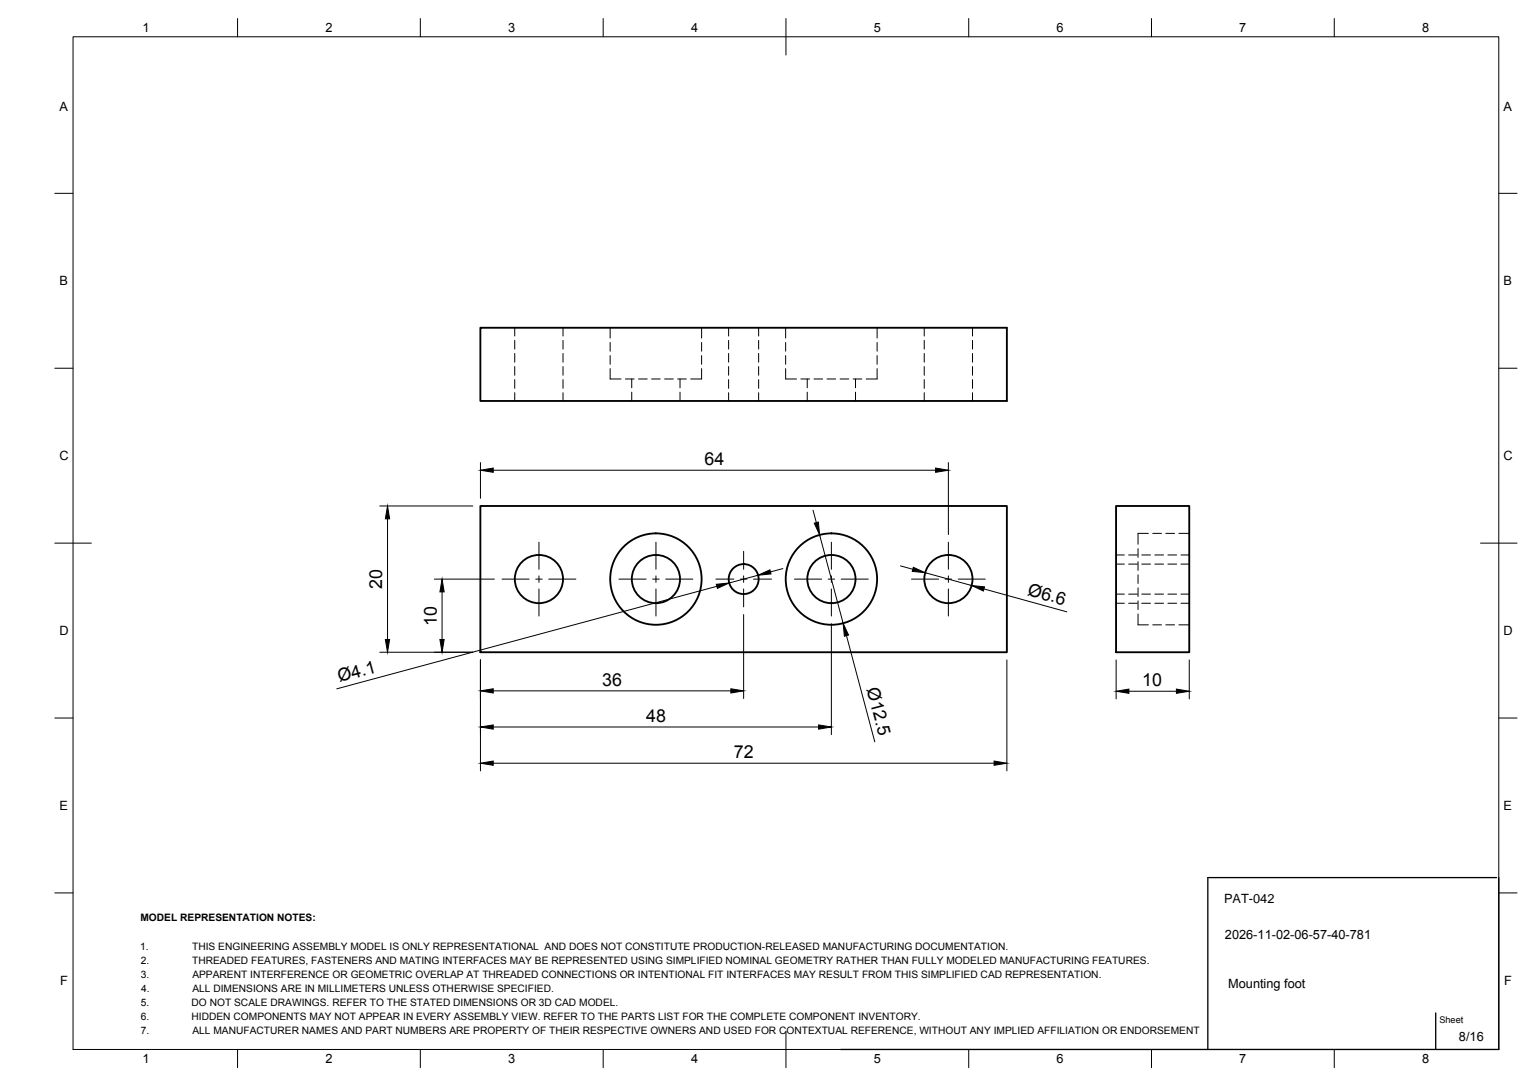
ISO-10303-21;
HEADER;
/* Generated by software containing ST-Developer
 * from STEP Tools, Inc. (www.steptools.com) 
 */

FILE_DESCRIPTION(
/* description */ ('Manifold and mounting hardware'),
/* implementation_level */ '2;1');

FILE_NAME(
/* name */ 'Mounting foot.step',
/* time_stamp */ '2026-10-28T21:46:49-07:00',
/* author */ (''),
/* organization */ (''),
/* preprocessor_version */ 'ST-DEVELOPER v20.2',
/* originating_system */ 'Autodesk Translation Framework v15.17.0.0',
/* authorisation */ '');

FILE_SCHEMA (('AUTOMOTIVE_DESIGN { 1 0 10303 214 3 1 1 }'));
ENDSEC;

DATA;
#10=MECHANICAL_DESIGN_GEOMETRIC_PRESENTATION_REPRESENTATION('',(#155),#5638);
#127=SHAPE_REPRESENTATION_RELATIONSHIP('SRR','None',#5706,#141);
#141=ADVANCED_BREP_SHAPE_REPRESENTATION('',(#169),#5628);
#155=STYLED_ITEM('',(#5853),#169);
#169=MANIFOLD_SOLID_BREP('Body1',#3145);
#212=FACE_BOUND('',#644,.T.);
#213=FACE_BOUND('',#647,.T.);
#214=FACE_BOUND('',#655,.T.);
#215=FACE_BOUND('',#656,.T.);
#216=FACE_BOUND('',#657,.T.);
#217=FACE_BOUND('',#658,.T.);
#218=FACE_BOUND('',#659,.T.);
#219=FACE_BOUND('',#661,.T.);
#220=FACE_BOUND('',#662,.T.);
#221=FACE_BOUND('',#663,.T.);
#222=FACE_BOUND('',#664,.T.);
#223=FACE_BOUND('',#665,.T.);
#300=CYLINDRICAL_SURFACE('',#3477,0.205);
#301=CYLINDRICAL_SURFACE('',#3480,0.33);
#302=CYLINDRICAL_SURFACE('',#3483,0.33);
#303=CYLINDRICAL_SURFACE('',#3486,0.625);
#304=CYLINDRICAL_SURFACE('',#3491,0.625);
#305=CYLINDRICAL_SURFACE('',#3496,0.33);
#306=CYLINDRICAL_SURFACE('',#3498,0.33);
#419=FACE_OUTER_BOUND('',#639,.T.);
#420=FACE_OUTER_BOUND('',#640,.T.);
#421=FACE_OUTER_BOUND('',#641,.T.);
#422=FACE_OUTER_BOUND('',#642,.T.);
#423=FACE_OUTER_BOUND('',#643,.T.);
#424=FACE_OUTER_BOUND('',#645,.T.);
#425=FACE_OUTER_BOUND('',#646,.T.);
#426=FACE_OUTER_BOUND('',#648,.T.);
#427=FACE_OUTER_BOUND('',#649,.T.);
#428=FACE_OUTER_BOUND('',#650,.T.);
#429=FACE_OUTER_BOUND('',#651,.T.);
#430=FACE_OUTER_BOUND('',#652,.T.);
#431=FACE_OUTER_BOUND('',#653,.T.);
#432=FACE_OUTER_BOUND('',#654,.T.);
#433=FACE_OUTER_BOUND('',#660,.T.);
#639=EDGE_LOOP('',(#2442,#2443,#2444,#2445));
#640=EDGE_LOOP('',(#2446,#2447,#2448,#2449));
#641=EDGE_LOOP('',(#2450,#2451,#2452,#2453));
#642=EDGE_LOOP('',(#2454,#2455,#2456,#2457));
#643=EDGE_LOOP('',(#2458));
#644=EDGE_LOOP('',(#2459));
#645=EDGE_LOOP('',(#2460,#2461,#2462,#2463));
#646=EDGE_LOOP('',(#2464));
#647=EDGE_LOOP('',(#2465));
#648=EDGE_LOOP('',(#2466,#2467,#2468,#2469));
#649=EDGE_LOOP('',(#2470,#2471,#2472,#2473));
#650=EDGE_LOOP('',(#2474,#2475,#2476,#2477));
#651=EDGE_LOOP('',(#2478,#2479,#2480,#2481));
#652=EDGE_LOOP('',(#2482,#2483,#2484,#2485));
#653=EDGE_LOOP('',(#2486,#2487,#2488,#2489));
#654=EDGE_LOOP('',(#2490,#2491,#2492,#2493));
#655=EDGE_LOOP('',(#2494));
#656=EDGE_LOOP('',(#2495));
#657=EDGE_LOOP('',(#2496));
#658=EDGE_LOOP('',(#2497));
#659=EDGE_LOOP('',(#2498));
#660=EDGE_LOOP('',(#2499,#2500,#2501,#2502));
#661=EDGE_LOOP('',(#2503));
#662=EDGE_LOOP('',(#2504));
#663=EDGE_LOOP('',(#2505));
#664=EDGE_LOOP('',(#2506));
#665=EDGE_LOOP('',(#2507));
#833=CIRCLE('',#3478,0.205);
#834=CIRCLE('',#3479,0.205);
#835=CIRCLE('',#3481,0.33);
#836=CIRCLE('',#3482,0.33);
#837=CIRCLE('',#3484,0.33);
#838=CIRCLE('',#3485,0.33);
#839=CIRCLE('',#3487,0.625);
#840=CIRCLE('',#3488,0.625);
#841=CIRCLE('',#3490,0.33);
#842=CIRCLE('',#3492,0.625);
#843=CIRCLE('',#3493,0.625);
#844=CIRCLE('',#3495,0.33);
#845=CIRCLE('',#3497,0.33);
#846=CIRCLE('',#3499,0.33);
#1020=LINE('',#5144,#1267);
#1021=LINE('',#5150,#1268);
#1022=LINE('',#5156,#1269);
#1023=LINE('',#5162,#1270);
#1024=LINE('',#5171,#1271);
#1025=LINE('',#5178,#1272);
#1026=LINE('',#5182,#1273);
#1027=LINE('',#5187,#1274);
#1028=LINE('',#5189,#1275);
#1029=LINE('',#5191,#1276);
#1030=LINE('',#5192,#1277);
#1031=LINE('',#5195,#1278);
#1032=LINE('',#5197,#1279);
#1033=LINE('',#5198,#1280);
#1034=LINE('',#5201,#1281);
#1035=LINE('',#5203,#1282);
#1036=LINE('',#5204,#1283);
#1037=LINE('',#5206,#1284);
#1038=LINE('',#5207,#1285);
#1267=VECTOR('',#4135,0.205);
#1268=VECTOR('',#4142,0.33);
#1269=VECTOR('',#4149,0.33);
#1270=VECTOR('',#4156,0.625);
#1271=VECTOR('',#4167,0.625);
#1272=VECTOR('',#4176,0.33);
#1273=VECTOR('',#4181,0.33);
#1274=VECTOR('',#4186,1.);
#1275=VECTOR('',#4187,1.);
#1276=VECTOR('',#4188,1.);
#1277=VECTOR('',#4189,1.);
#1278=VECTOR('',#4192,1.);
#1279=VECTOR('',#4193,1.);
#1280=VECTOR('',#4194,1.);
#1281=VECTOR('',#4197,1.);
#1282=VECTOR('',#4198,1.);
#1283=VECTOR('',#4199,1.);
#1284=VECTOR('',#4202,1.);
#1285=VECTOR('',#4203,1.);
#1523=VERTEX_POINT('',#5141);
#1524=VERTEX_POINT('',#5143);
#1525=VERTEX_POINT('',#5147);
#1526=VERTEX_POINT('',#5149);
#1527=VERTEX_POINT('',#5153);
#1528=VERTEX_POINT('',#5155);
#1529=VERTEX_POINT('',#5159);
#1530=VERTEX_POINT('',#5161);
#1531=VERTEX_POINT('',#5165);
#1532=VERTEX_POINT('',#5168);
#1533=VERTEX_POINT('',#5170);
#1534=VERTEX_POINT('',#5174);
#1535=VERTEX_POINT('',#5177);
#1536=VERTEX_POINT('',#5181);
#1537=VERTEX_POINT('',#5185);
#1538=VERTEX_POINT('',#5186);
#1539=VERTEX_POINT('',#5188);
#1540=VERTEX_POINT('',#5190);
#1541=VERTEX_POINT('',#5194);
#1542=VERTEX_POINT('',#5196);
#1543=VERTEX_POINT('',#5200);
#1544=VERTEX_POINT('',#5202);
#1850=EDGE_CURVE('',#1523,#1523,#833,.T.);
#1851=EDGE_CURVE('',#1523,#1524,#1020,.T.);
#1852=EDGE_CURVE('',#1524,#1524,#834,.T.);
#1853=EDGE_CURVE('',#1525,#1525,#835,.T.);
#1854=EDGE_CURVE('',#1525,#1526,#1021,.T.);
#1855=EDGE_CURVE('',#1526,#1526,#836,.T.);
#1856=EDGE_CURVE('',#1527,#1527,#837,.T.);
#1857=EDGE_CURVE('',#1527,#1528,#1022,.T.);
#1858=EDGE_CURVE('',#1528,#1528,#838,.T.);
#1859=EDGE_CURVE('',#1529,#1529,#839,.T.);
#1860=EDGE_CURVE('',#1529,#1530,#1023,.T.);
#1861=EDGE_CURVE('',#1530,#1530,#840,.T.);
#1862=EDGE_CURVE('',#1531,#1531,#841,.T.);
#1863=EDGE_CURVE('',#1532,#1532,#842,.T.);
#1864=EDGE_CURVE('',#1532,#1533,#1024,.T.);
#1865=EDGE_CURVE('',#1533,#1533,#843,.T.);
#1866=EDGE_CURVE('',#1534,#1534,#844,.T.);
#1867=EDGE_CURVE('',#1531,#1535,#1025,.T.);
#1868=EDGE_CURVE('',#1535,#1535,#845,.T.);
#1869=EDGE_CURVE('',#1534,#1536,#1026,.T.);
#1870=EDGE_CURVE('',#1536,#1536,#846,.T.);
#1871=EDGE_CURVE('',#1537,#1538,#1027,.T.);
#1872=EDGE_CURVE('',#1538,#1539,#1028,.T.);
#1873=EDGE_CURVE('',#1540,#1539,#1029,.T.);
#1874=EDGE_CURVE('',#1537,#1540,#1030,.T.);
#1875=EDGE_CURVE('',#1541,#1537,#1031,.T.);
#1876=EDGE_CURVE('',#1542,#1540,#1032,.T.);
#1877=EDGE_CURVE('',#1541,#1542,#1033,.T.);
#1878=EDGE_CURVE('',#1543,#1541,#1034,.T.);
#1879=EDGE_CURVE('',#1544,#1542,#1035,.T.);
#1880=EDGE_CURVE('',#1543,#1544,#1036,.T.);
#1881=EDGE_CURVE('',#1538,#1543,#1037,.T.);
#1882=EDGE_CURVE('',#1539,#1544,#1038,.T.);
#2442=ORIENTED_EDGE('',*,*,#1850,.F.);
#2443=ORIENTED_EDGE('',*,*,#1851,.T.);
#2444=ORIENTED_EDGE('',*,*,#1852,.F.);
#2445=ORIENTED_EDGE('',*,*,#1851,.F.);
#2446=ORIENTED_EDGE('',*,*,#1853,.F.);
#2447=ORIENTED_EDGE('',*,*,#1854,.T.);
#2448=ORIENTED_EDGE('',*,*,#1855,.F.);
#2449=ORIENTED_EDGE('',*,*,#1854,.F.);
#2450=ORIENTED_EDGE('',*,*,#1856,.F.);
#2451=ORIENTED_EDGE('',*,*,#1857,.T.);
#2452=ORIENTED_EDGE('',*,*,#1858,.F.);
#2453=ORIENTED_EDGE('',*,*,#1857,.F.);
#2454=ORIENTED_EDGE('',*,*,#1859,.F.);
#2455=ORIENTED_EDGE('',*,*,#1860,.T.);
#2456=ORIENTED_EDGE('',*,*,#1861,.T.);
#2457=ORIENTED_EDGE('',*,*,#1860,.F.);
#2458=ORIENTED_EDGE('',*,*,#1861,.F.);
#2459=ORIENTED_EDGE('',*,*,#1862,.F.);
#2460=ORIENTED_EDGE('',*,*,#1863,.F.);
#2461=ORIENTED_EDGE('',*,*,#1864,.T.);
#2462=ORIENTED_EDGE('',*,*,#1865,.T.);
#2463=ORIENTED_EDGE('',*,*,#1864,.F.);
#2464=ORIENTED_EDGE('',*,*,#1865,.F.);
#2465=ORIENTED_EDGE('',*,*,#1866,.F.);
#2466=ORIENTED_EDGE('',*,*,#1862,.T.);
#2467=ORIENTED_EDGE('',*,*,#1867,.T.);
#2468=ORIENTED_EDGE('',*,*,#1868,.F.);
#2469=ORIENTED_EDGE('',*,*,#1867,.F.);
#2470=ORIENTED_EDGE('',*,*,#1866,.T.);
#2471=ORIENTED_EDGE('',*,*,#1869,.T.);
#2472=ORIENTED_EDGE('',*,*,#1870,.F.);
#2473=ORIENTED_EDGE('',*,*,#1869,.F.);
#2474=ORIENTED_EDGE('',*,*,#1871,.T.);
#2475=ORIENTED_EDGE('',*,*,#1872,.T.);
#2476=ORIENTED_EDGE('',*,*,#1873,.F.);
#2477=ORIENTED_EDGE('',*,*,#1874,.F.);
#2478=ORIENTED_EDGE('',*,*,#1875,.T.);
#2479=ORIENTED_EDGE('',*,*,#1874,.T.);
#2480=ORIENTED_EDGE('',*,*,#1876,.F.);
#2481=ORIENTED_EDGE('',*,*,#1877,.F.);
#2482=ORIENTED_EDGE('',*,*,#1878,.T.);
#2483=ORIENTED_EDGE('',*,*,#1877,.T.);
#2484=ORIENTED_EDGE('',*,*,#1879,.F.);
#2485=ORIENTED_EDGE('',*,*,#1880,.F.);
#2486=ORIENTED_EDGE('',*,*,#1881,.T.);
#2487=ORIENTED_EDGE('',*,*,#1880,.T.);
#2488=ORIENTED_EDGE('',*,*,#1882,.F.);
#2489=ORIENTED_EDGE('',*,*,#1872,.F.);
#2490=ORIENTED_EDGE('',*,*,#1882,.T.);
#2491=ORIENTED_EDGE('',*,*,#1879,.T.);
#2492=ORIENTED_EDGE('',*,*,#1876,.T.);
#2493=ORIENTED_EDGE('',*,*,#1873,.T.);
#2494=ORIENTED_EDGE('',*,*,#1852,.T.);
#2495=ORIENTED_EDGE('',*,*,#1855,.T.);
#2496=ORIENTED_EDGE('',*,*,#1858,.T.);
#2497=ORIENTED_EDGE('',*,*,#1868,.T.);
#2498=ORIENTED_EDGE('',*,*,#1870,.T.);
#2499=ORIENTED_EDGE('',*,*,#1881,.F.);
#2500=ORIENTED_EDGE('',*,*,#1871,.F.);
#2501=ORIENTED_EDGE('',*,*,#1875,.F.);
#2502=ORIENTED_EDGE('',*,*,#1878,.F.);
#2503=ORIENTED_EDGE('',*,*,#1850,.T.);
#2504=ORIENTED_EDGE('',*,*,#1853,.T.);
#2505=ORIENTED_EDGE('',*,*,#1856,.T.);
#2506=ORIENTED_EDGE('',*,*,#1859,.T.);
#2507=ORIENTED_EDGE('',*,*,#1863,.T.);
#2892=PLANE('',#3489);
#2893=PLANE('',#3494);
#2894=PLANE('',#3500);
#2895=PLANE('',#3501);
#2896=PLANE('',#3502);
#2897=PLANE('',#3503);
#2898=PLANE('',#3504);
#2899=PLANE('',#3505);
#3043=ADVANCED_FACE('',(#419),#300,.F.);
#3044=ADVANCED_FACE('',(#420),#301,.F.);
#3045=ADVANCED_FACE('',(#421),#302,.F.);
#3046=ADVANCED_FACE('',(#422),#303,.F.);
#3047=ADVANCED_FACE('',(#423,#212),#2892,.F.);
#3048=ADVANCED_FACE('',(#424),#304,.F.);
#3049=ADVANCED_FACE('',(#425,#213),#2893,.F.);
#3050=ADVANCED_FACE('',(#426),#305,.F.);
#3051=ADVANCED_FACE('',(#427),#306,.F.);
#3052=ADVANCED_FACE('',(#428),#2894,.T.);
#3053=ADVANCED_FACE('',(#429),#2895,.T.);
#3054=ADVANCED_FACE('',(#430),#2896,.T.);
#3055=ADVANCED_FACE('',(#431),#2897,.T.);
#3056=ADVANCED_FACE('',(#432,#214,#215,#216,#217,#218),#2898,.T.);
#3057=ADVANCED_FACE('',(#433,#219,#220,#221,#222,#223),#2899,.F.);
#3145=CLOSED_SHELL('',(#3043,#3044,#3045,#3046,#3047,#3048,#3049,#3050,
#3051,#3052,#3053,#3054,#3055,#3056,#3057));
#3476=AXIS2_PLACEMENT_3D('',#5139,#4129,#4130);
#3477=AXIS2_PLACEMENT_3D('',#5140,#4131,#4132);
#3478=AXIS2_PLACEMENT_3D('',#5142,#4133,#4134);
#3479=AXIS2_PLACEMENT_3D('',#5145,#4136,#4137);
#3480=AXIS2_PLACEMENT_3D('',#5146,#4138,#4139);
#3481=AXIS2_PLACEMENT_3D('',#5148,#4140,#4141);
#3482=AXIS2_PLACEMENT_3D('',#5151,#4143,#4144);
#3483=AXIS2_PLACEMENT_3D('',#5152,#4145,#4146);
#3484=AXIS2_PLACEMENT_3D('',#5154,#4147,#4148);
#3485=AXIS2_PLACEMENT_3D('',#5157,#4150,#4151);
#3486=AXIS2_PLACEMENT_3D('',#5158,#4152,#4153);
#3487=AXIS2_PLACEMENT_3D('',#5160,#4154,#4155);
#3488=AXIS2_PLACEMENT_3D('',#5163,#4157,#4158);
#3489=AXIS2_PLACEMENT_3D('',#5164,#4159,#4160);
#3490=AXIS2_PLACEMENT_3D('',#5166,#4161,#4162);
#3491=AXIS2_PLACEMENT_3D('',#5167,#4163,#4164);
#3492=AXIS2_PLACEMENT_3D('',#5169,#4165,#4166);
#3493=AXIS2_PLACEMENT_3D('',#5172,#4168,#4169);
#3494=AXIS2_PLACEMENT_3D('',#5173,#4170,#4171);
#3495=AXIS2_PLACEMENT_3D('',#5175,#4172,#4173);
#3496=AXIS2_PLACEMENT_3D('',#5176,#4174,#4175);
#3497=AXIS2_PLACEMENT_3D('',#5179,#4177,#4178);
#3498=AXIS2_PLACEMENT_3D('',#5180,#4179,#4180);
#3499=AXIS2_PLACEMENT_3D('',#5183,#4182,#4183);
#3500=AXIS2_PLACEMENT_3D('',#5184,#4184,#4185);
#3501=AXIS2_PLACEMENT_3D('',#5193,#4190,#4191);
#3502=AXIS2_PLACEMENT_3D('',#5199,#4195,#4196);
#3503=AXIS2_PLACEMENT_3D('',#5205,#4200,#4201);
#3504=AXIS2_PLACEMENT_3D('',#5208,#4204,#4205);
#3505=AXIS2_PLACEMENT_3D('',#5209,#4206,#4207);
#4129=DIRECTION('axis',(0.,0.,1.));
#4130=DIRECTION('refdir',(1.,0.,0.));
#4131=DIRECTION('center_axis',(0.,0.,1.));
#4132=DIRECTION('ref_axis',(1.,0.,0.));
#4133=DIRECTION('center_axis',(0.,0.,1.));
#4134=DIRECTION('ref_axis',(1.,0.,0.));
#4135=DIRECTION('',(0.,0.,1.));
#4136=DIRECTION('center_axis',(0.,0.,-1.));
#4137=DIRECTION('ref_axis',(1.,0.,0.));
#4138=DIRECTION('center_axis',(0.,0.,1.));
#4139=DIRECTION('ref_axis',(1.,0.,0.));
#4140=DIRECTION('center_axis',(0.,0.,1.));
#4141=DIRECTION('ref_axis',(1.,0.,0.));
#4142=DIRECTION('',(0.,0.,1.));
#4143=DIRECTION('center_axis',(0.,0.,-1.));
#4144=DIRECTION('ref_axis',(1.,0.,0.));
#4145=DIRECTION('center_axis',(0.,0.,1.));
#4146=DIRECTION('ref_axis',(1.,0.,0.));
#4147=DIRECTION('center_axis',(0.,0.,1.));
#4148=DIRECTION('ref_axis',(1.,0.,0.));
#4149=DIRECTION('',(0.,0.,1.));
#4150=DIRECTION('center_axis',(0.,0.,-1.));
#4151=DIRECTION('ref_axis',(1.,0.,0.));
#4152=DIRECTION('center_axis',(0.,0.,1.));
#4153=DIRECTION('ref_axis',(1.,0.,0.));
#4154=DIRECTION('center_axis',(0.,0.,1.));
#4155=DIRECTION('ref_axis',(1.,0.,0.));
#4156=DIRECTION('',(0.,0.,1.));
#4157=DIRECTION('center_axis',(0.,0.,1.));
#4158=DIRECTION('ref_axis',(1.,0.,0.));
#4159=DIRECTION('center_axis',(0.,0.,1.));
#4160=DIRECTION('ref_axis',(1.,0.,0.));
#4161=DIRECTION('center_axis',(0.,0.,-1.));
#4162=DIRECTION('ref_axis',(1.,0.,0.));
#4163=DIRECTION('center_axis',(0.,0.,1.));
#4164=DIRECTION('ref_axis',(1.,0.,0.));
#4165=DIRECTION('center_axis',(0.,0.,1.));
#4166=DIRECTION('ref_axis',(1.,0.,0.));
#4167=DIRECTION('',(0.,0.,1.));
#4168=DIRECTION('center_axis',(0.,0.,1.));
#4169=DIRECTION('ref_axis',(1.,0.,0.));
#4170=DIRECTION('center_axis',(0.,0.,1.));
#4171=DIRECTION('ref_axis',(1.,0.,0.));
#4172=DIRECTION('center_axis',(0.,0.,-1.));
#4173=DIRECTION('ref_axis',(1.,0.,0.));
#4174=DIRECTION('center_axis',(0.,0.,1.));
#4175=DIRECTION('ref_axis',(1.,0.,0.));
#4176=DIRECTION('',(0.,0.,1.));
#4177=DIRECTION('center_axis',(0.,0.,-1.));
#4178=DIRECTION('ref_axis',(1.,0.,0.));
#4179=DIRECTION('center_axis',(0.,0.,1.));
#4180=DIRECTION('ref_axis',(1.,0.,0.));
#4181=DIRECTION('',(0.,0.,1.));
#4182=DIRECTION('center_axis',(0.,0.,-1.));
#4183=DIRECTION('ref_axis',(1.,0.,0.));
#4184=DIRECTION('center_axis',(0.,1.,0.));
#4185=DIRECTION('ref_axis',(-1.,0.,0.));
#4186=DIRECTION('',(-1.,0.,0.));
#4187=DIRECTION('',(0.,0.,1.));
#4188=DIRECTION('',(-1.,0.,0.));
#4189=DIRECTION('',(0.,0.,1.));
#4190=DIRECTION('center_axis',(1.,0.,0.));
#4191=DIRECTION('ref_axis',(0.,1.,0.));
#4192=DIRECTION('',(0.,1.,0.));
#4193=DIRECTION('',(0.,1.,0.));
#4194=DIRECTION('',(0.,0.,1.));
#4195=DIRECTION('center_axis',(0.,-1.,0.));
#4196=DIRECTION('ref_axis',(1.,0.,0.));
#4197=DIRECTION('',(1.,0.,0.));
#4198=DIRECTION('',(1.,0.,0.));
#4199=DIRECTION('',(0.,0.,1.));
#4200=DIRECTION('center_axis',(-1.,0.,0.));
#4201=DIRECTION('ref_axis',(0.,-1.,0.));
#4202=DIRECTION('',(0.,-1.,0.));
#4203=DIRECTION('',(0.,-1.,0.));
#4204=DIRECTION('center_axis',(0.,0.,1.));
#4205=DIRECTION('ref_axis',(1.,0.,0.));
#4206=DIRECTION('center_axis',(0.,0.,1.));
#4207=DIRECTION('ref_axis',(1.,0.,0.));
#5139=CARTESIAN_POINT('',(0.,0.,0.));
#5140=CARTESIAN_POINT('Origin',(-4.5,0.,0.9));
#5141=CARTESIAN_POINT('',(-4.705,-2.51052593825207E-17,1.));
#5142=CARTESIAN_POINT('Origin',(-4.5,0.,1.));
#5143=CARTESIAN_POINT('',(-4.705,2.51052593825207E-17,2.));
#5144=CARTESIAN_POINT('',(-4.705,-2.51052593825207E-17,0.9));
#5145=CARTESIAN_POINT('Origin',(-4.5,0.,2.));
#5146=CARTESIAN_POINT('Origin',(-4.5,-2.8,0.9));
#5147=CARTESIAN_POINT('',(-4.83,-2.8,1.));
#5148=CARTESIAN_POINT('Origin',(-4.5,-2.8,1.));
#5149=CARTESIAN_POINT('',(-4.83,-2.8,2.));
#5150=CARTESIAN_POINT('',(-4.83,-2.8,0.9));
#5151=CARTESIAN_POINT('Origin',(-4.5,-2.8,2.));
#5152=CARTESIAN_POINT('Origin',(-4.5,2.8,0.9));
#5153=CARTESIAN_POINT('',(-4.83,2.8,1.));
#5154=CARTESIAN_POINT('Origin',(-4.5,2.8,1.));
#5155=CARTESIAN_POINT('',(-4.83,2.8,2.));
#5156=CARTESIAN_POINT('',(-4.83,2.8,0.9));
#5157=CARTESIAN_POINT('Origin',(-4.5,2.8,2.));
#5158=CARTESIAN_POINT('Origin',(-4.5,-1.2,0.9));
#5159=CARTESIAN_POINT('',(-5.125,-1.2,1.));
#5160=CARTESIAN_POINT('Origin',(-4.5,-1.2,1.));
#5161=CARTESIAN_POINT('',(-5.125,-1.2,1.7));
#5162=CARTESIAN_POINT('',(-5.125,-1.2,0.9));
#5163=CARTESIAN_POINT('Origin',(-4.5,-1.2,1.7));
#5164=CARTESIAN_POINT('Origin',(-4.5,-1.2,1.7));
#5165=CARTESIAN_POINT('',(-4.83,-1.2,1.7));
#5166=CARTESIAN_POINT('Origin',(-4.5,-1.2,1.7));
#5167=CARTESIAN_POINT('Origin',(-4.5,1.2,0.9));
#5168=CARTESIAN_POINT('',(-5.125,1.2,1.));
#5169=CARTESIAN_POINT('Origin',(-4.5,1.2,1.));
#5170=CARTESIAN_POINT('',(-5.125,1.2,1.7));
#5171=CARTESIAN_POINT('',(-5.125,1.2,0.9));
#5172=CARTESIAN_POINT('Origin',(-4.5,1.2,1.7));
#5173=CARTESIAN_POINT('Origin',(-4.5,1.2,1.7));
#5174=CARTESIAN_POINT('',(-4.83,1.2,1.7));
#5175=CARTESIAN_POINT('Origin',(-4.5,1.2,1.7));
#5176=CARTESIAN_POINT('Origin',(-4.5,-1.2,0.9));
#5177=CARTESIAN_POINT('',(-4.83,-1.2,2.));
#5178=CARTESIAN_POINT('',(-4.83,-1.2,0.9));
#5179=CARTESIAN_POINT('Origin',(-4.5,-1.2,2.));
#5180=CARTESIAN_POINT('Origin',(-4.5,1.2,0.9));
#5181=CARTESIAN_POINT('',(-4.83,1.2,2.));
#5182=CARTESIAN_POINT('',(-4.83,1.2,0.9));
#5183=CARTESIAN_POINT('Origin',(-4.5,1.2,2.));
#5184=CARTESIAN_POINT('Origin',(-3.5,3.6,1.));
#5185=CARTESIAN_POINT('',(-3.5,3.6,1.));
#5186=CARTESIAN_POINT('',(-5.5,3.6,1.));
#5187=CARTESIAN_POINT('',(-3.5,3.6,1.));
#5188=CARTESIAN_POINT('',(-5.5,3.6,2.));
#5189=CARTESIAN_POINT('',(-5.5,3.6,1.));
#5190=CARTESIAN_POINT('',(-3.5,3.6,2.));
#5191=CARTESIAN_POINT('',(-3.5,3.6,2.));
#5192=CARTESIAN_POINT('',(-3.5,3.6,1.));
#5193=CARTESIAN_POINT('Origin',(-3.5,-3.6,1.));
#5194=CARTESIAN_POINT('',(-3.5,-3.6,1.));
#5195=CARTESIAN_POINT('',(-3.5,-3.6,1.));
#5196=CARTESIAN_POINT('',(-3.5,-3.6,2.));
#5197=CARTESIAN_POINT('',(-3.5,-3.6,2.));
#5198=CARTESIAN_POINT('',(-3.5,-3.6,1.));
#5199=CARTESIAN_POINT('Origin',(-5.5,-3.6,1.));
#5200=CARTESIAN_POINT('',(-5.5,-3.6,1.));
#5201=CARTESIAN_POINT('',(-5.5,-3.6,1.));
#5202=CARTESIAN_POINT('',(-5.5,-3.6,2.));
#5203=CARTESIAN_POINT('',(-5.5,-3.6,2.));
#5204=CARTESIAN_POINT('',(-5.5,-3.6,1.));
#5205=CARTESIAN_POINT('Origin',(-5.5,3.6,1.));
#5206=CARTESIAN_POINT('',(-5.5,3.6,1.));
#5207=CARTESIAN_POINT('',(-5.5,3.6,2.));
#5208=CARTESIAN_POINT('Origin',(-4.5,0.,2.));
#5209=CARTESIAN_POINT('Origin',(-4.5,0.,1.));
#5611=UNCERTAINTY_MEASURE_WITH_UNIT(LENGTH_MEASURE(0.001),#5639,
'DISTANCE_ACCURACY_VALUE',
'Maximum model space distance between geometric entities at asserted c
onnectivities');
#5621=UNCERTAINTY_MEASURE_WITH_UNIT(LENGTH_MEASURE(0.001),#5639,
'DISTANCE_ACCURACY_VALUE',
'Maximum model space distance between geometric entities at asserted c
onnectivities');
#5628=(
GEOMETRIC_REPRESENTATION_CONTEXT(3)
GLOBAL_UNCERTAINTY_ASSIGNED_CONTEXT((#5611))
GLOBAL_UNIT_ASSIGNED_CONTEXT((#5639,#5641,#5642))
REPRESENTATION_CONTEXT('','3D')
);
#5638=(
GEOMETRIC_REPRESENTATION_CONTEXT(3)
GLOBAL_UNCERTAINTY_ASSIGNED_CONTEXT((#5621))
GLOBAL_UNIT_ASSIGNED_CONTEXT((#5639,#5641,#5642))
REPRESENTATION_CONTEXT('','3D')
);
#5639=(
LENGTH_UNIT()
NAMED_UNIT(*)
SI_UNIT(.CENTI.,.METRE.)
);
#5641=(
NAMED_UNIT(*)
PLANE_ANGLE_UNIT()
SI_UNIT($,.RADIAN.)
);
#5642=(
NAMED_UNIT(*)
SI_UNIT($,.STERADIAN.)
SOLID_ANGLE_UNIT()
);
#5649=SHAPE_DEFINITION_REPRESENTATION(#5665,#5706);
#5665=PRODUCT_DEFINITION_SHAPE('',$,#5723);
#5706=SHAPE_REPRESENTATION('',(#3476),#5628);
#5716=PRODUCT_DEFINITION_CONTEXT('part definition',#5766,'design');
#5723=PRODUCT_DEFINITION('Mounting foot','Mounting foot',#5739,
#5716);
#5739=PRODUCT_DEFINITION_FORMATION('',$,#5774);
#5766=APPLICATION_CONTEXT(
'Core Data for Automotive Mechanical Design Process');
#5767=PRODUCT_CONTEXT('part definition',#5766,'mechanical');
#5774=PRODUCT('Mounting foot','Mounting foot',
'Mounting foot',(#5767));
#5847=COLOUR_RGB('Sky Blue',0.24,0.69,0.87);
#5848=FILL_AREA_STYLE_COLOUR('',#5847);
#5849=FILL_AREA_STYLE('',(#5848));
#5850=SURFACE_STYLE_FILL_AREA(#5849);
#5851=SURFACE_SIDE_STYLE('',(#5850));
#5852=SURFACE_STYLE_USAGE(.BOTH.,#5851);
#5853=PRESENTATION_STYLE_ASSIGNMENT((#5852));
ENDSEC;
END-ISO-10303-21;
